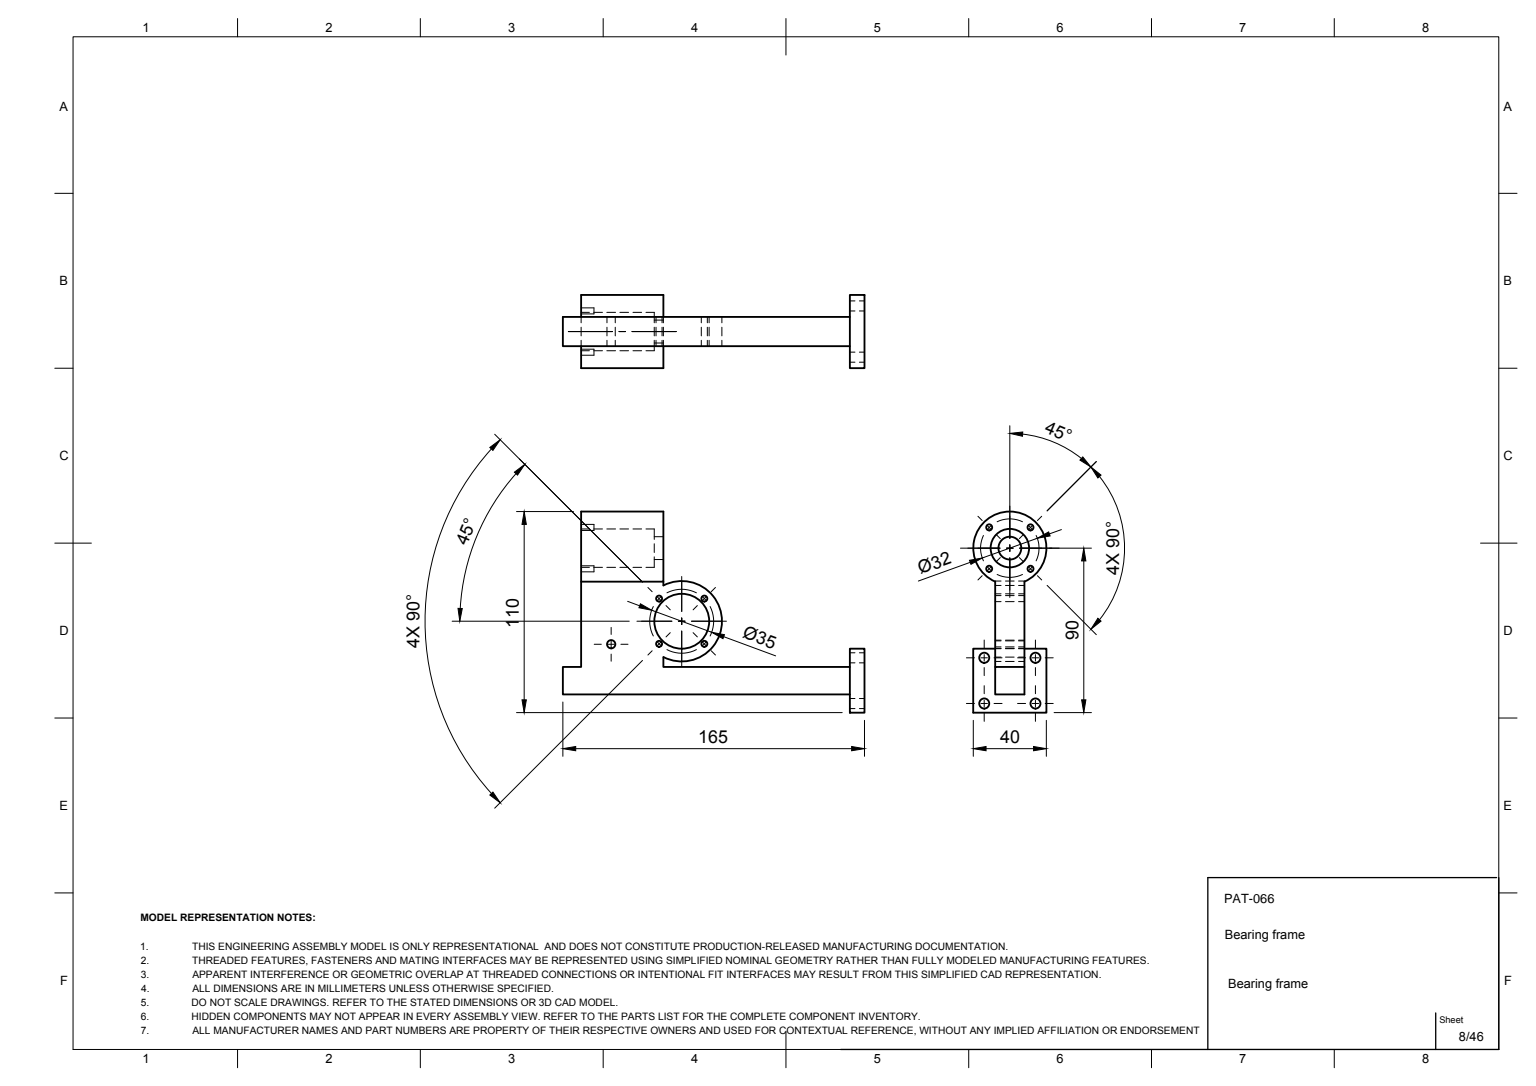
ISO-10303-21;
HEADER;
/* Generated by software containing ST-Developer
 * from STEP Tools, Inc. (www.steptools.com) 
 */

FILE_DESCRIPTION(
/* description */ ('Lever-operated bar clamp (toggle)'),
/* implementation_level */ '2;1');

FILE_NAME(
/* name */ 'Bearing frame.step',
/* time_stamp */ '2026-10-28T03:25:02-07:00',
/* author */ (''),
/* organization */ (''),
/* preprocessor_version */ 'ST-DEVELOPER v20.2',
/* originating_system */ 'Autodesk Translation Framework v15.17.0.0',
/* authorisation */ '');

FILE_SCHEMA (('AUTOMOTIVE_DESIGN { 1 0 10303 214 3 1 1 }'));
ENDSEC;

DATA;
#10=MECHANICAL_DESIGN_GEOMETRIC_PRESENTATION_REPRESENTATION('',(#413),#12413);
#337=SHAPE_REPRESENTATION_RELATIONSHIP('SRR','None',#12576,#375);
#375=ADVANCED_BREP_SHAPE_REPRESENTATION('',(#460),#12373);
#413=STYLED_ITEM('',(#12869),#460);
#460=MANIFOLD_SOLID_BREP('Body1',#6572);
#516=FACE_BOUND('',#1355,.T.);
#517=FACE_BOUND('',#1360,.T.);
#518=FACE_BOUND('',#1361,.T.);
#519=FACE_BOUND('',#1362,.T.);
#520=FACE_BOUND('',#1363,.T.);
#521=FACE_BOUND('',#1364,.T.);
#522=FACE_BOUND('',#1365,.T.);
#523=FACE_BOUND('',#1367,.T.);
#524=FACE_BOUND('',#1368,.T.);
#525=FACE_BOUND('',#1369,.T.);
#526=FACE_BOUND('',#1370,.T.);
#527=FACE_BOUND('',#1371,.T.);
#528=FACE_BOUND('',#1373,.T.);
#529=FACE_BOUND('',#1374,.T.);
#530=FACE_BOUND('',#1375,.T.);
#531=FACE_BOUND('',#1376,.T.);
#532=FACE_BOUND('',#1377,.T.);
#533=FACE_BOUND('',#1385,.T.);
#534=FACE_BOUND('',#1386,.T.);
#535=FACE_BOUND('',#1387,.T.);
#536=FACE_BOUND('',#1388,.T.);
#537=FACE_BOUND('',#1389,.T.);
#538=FACE_BOUND('',#1390,.T.);
#539=FACE_BOUND('',#1393,.T.);
#540=FACE_BOUND('',#1398,.T.);
#541=FACE_BOUND('',#1399,.T.);
#542=FACE_BOUND('',#1400,.T.);
#543=FACE_BOUND('',#1401,.T.);
#669=PLANE('',#7093);
#670=PLANE('',#7097);
#671=PLANE('',#7101);
#672=PLANE('',#7105);
#673=PLANE('',#7133);
#674=PLANE('',#7143);
#675=PLANE('',#7145);
#676=PLANE('',#7146);
#677=PLANE('',#7147);
#678=PLANE('',#7148);
#679=PLANE('',#7149);
#680=PLANE('',#7150);
#681=PLANE('',#7151);
#682=PLANE('',#7154);
#683=PLANE('',#7155);
#684=PLANE('',#7156);
#685=PLANE('',#7157);
#686=PLANE('',#7158);
#687=PLANE('',#7159);
#688=PLANE('',#7160);
#914=FACE_OUTER_BOUND('',#1336,.T.);
#915=FACE_OUTER_BOUND('',#1337,.T.);
#916=FACE_OUTER_BOUND('',#1338,.T.);
#917=FACE_OUTER_BOUND('',#1339,.T.);
#918=FACE_OUTER_BOUND('',#1340,.T.);
#919=FACE_OUTER_BOUND('',#1341,.T.);
#920=FACE_OUTER_BOUND('',#1342,.T.);
#921=FACE_OUTER_BOUND('',#1343,.T.);
#922=FACE_OUTER_BOUND('',#1344,.T.);
#923=FACE_OUTER_BOUND('',#1345,.T.);
#924=FACE_OUTER_BOUND('',#1346,.T.);
#925=FACE_OUTER_BOUND('',#1347,.T.);
#926=FACE_OUTER_BOUND('',#1348,.T.);
#927=FACE_OUTER_BOUND('',#1349,.T.);
#928=FACE_OUTER_BOUND('',#1350,.T.);
#929=FACE_OUTER_BOUND('',#1351,.T.);
#930=FACE_OUTER_BOUND('',#1352,.T.);
#931=FACE_OUTER_BOUND('',#1353,.T.);
#932=FACE_OUTER_BOUND('',#1354,.T.);
#933=FACE_OUTER_BOUND('',#1356,.T.);
#934=FACE_OUTER_BOUND('',#1357,.T.);
#935=FACE_OUTER_BOUND('',#1358,.T.);
#936=FACE_OUTER_BOUND('',#1359,.T.);
#937=FACE_OUTER_BOUND('',#1366,.T.);
#938=FACE_OUTER_BOUND('',#1372,.T.);
#939=FACE_OUTER_BOUND('',#1378,.T.);
#940=FACE_OUTER_BOUND('',#1379,.T.);
#941=FACE_OUTER_BOUND('',#1380,.T.);
#942=FACE_OUTER_BOUND('',#1381,.T.);
#943=FACE_OUTER_BOUND('',#1382,.T.);
#944=FACE_OUTER_BOUND('',#1383,.T.);
#945=FACE_OUTER_BOUND('',#1384,.T.);
#946=FACE_OUTER_BOUND('',#1391,.T.);
#947=FACE_OUTER_BOUND('',#1392,.T.);
#948=FACE_OUTER_BOUND('',#1394,.T.);
#949=FACE_OUTER_BOUND('',#1395,.T.);
#950=FACE_OUTER_BOUND('',#1396,.T.);
#951=FACE_OUTER_BOUND('',#1397,.T.);
#1336=EDGE_LOOP('',(#4541,#4542,#4543,#4544));
#1337=EDGE_LOOP('',(#4545,#4546,#4547,#4548));
#1338=EDGE_LOOP('',(#4549));
#1339=EDGE_LOOP('',(#4550,#4551,#4552,#4553));
#1340=EDGE_LOOP('',(#4554));
#1341=EDGE_LOOP('',(#4555,#4556,#4557,#4558));
#1342=EDGE_LOOP('',(#4559));
#1343=EDGE_LOOP('',(#4560,#4561,#4562,#4563));
#1344=EDGE_LOOP('',(#4564));
#1345=EDGE_LOOP('',(#4565,#4566,#4567,#4568));
#1346=EDGE_LOOP('',(#4569,#4570,#4571,#4572));
#1347=EDGE_LOOP('',(#4573,#4574,#4575,#4576));
#1348=EDGE_LOOP('',(#4577,#4578,#4579,#4580));
#1349=EDGE_LOOP('',(#4581,#4582,#4583,#4584));
#1350=EDGE_LOOP('',(#4585,#4586,#4587,#4588));
#1351=EDGE_LOOP('',(#4589,#4590,#4591,#4592));
#1352=EDGE_LOOP('',(#4593,#4594,#4595,#4596));
#1353=EDGE_LOOP('',(#4597,#4598,#4599,#4600));
#1354=EDGE_LOOP('',(#4601));
#1355=EDGE_LOOP('',(#4602));
#1356=EDGE_LOOP('',(#4603,#4604,#4605,#4606));
#1357=EDGE_LOOP('',(#4607,#4608,#4609,#4610));
#1358=EDGE_LOOP('',(#4611,#4612,#4613,#4614));
#1359=EDGE_LOOP('',(#4615,#4616,#4617,#4618,#4619,#4620,#4621,#4622,#4623,
#4624));
#1360=EDGE_LOOP('',(#4625));
#1361=EDGE_LOOP('',(#4626));
#1362=EDGE_LOOP('',(#4627));
#1363=EDGE_LOOP('',(#4628));
#1364=EDGE_LOOP('',(#4629));
#1365=EDGE_LOOP('',(#4630));
#1366=EDGE_LOOP('',(#4631,#4632,#4633,#4634));
#1367=EDGE_LOOP('',(#4635));
#1368=EDGE_LOOP('',(#4636));
#1369=EDGE_LOOP('',(#4637));
#1370=EDGE_LOOP('',(#4638));
#1371=EDGE_LOOP('',(#4639));
#1372=EDGE_LOOP('',(#4640,#4641,#4642,#4643));
#1373=EDGE_LOOP('',(#4644,#4645,#4646,#4647));
#1374=EDGE_LOOP('',(#4648));
#1375=EDGE_LOOP('',(#4649));
#1376=EDGE_LOOP('',(#4650));
#1377=EDGE_LOOP('',(#4651));
#1378=EDGE_LOOP('',(#4652,#4653,#4654,#4655));
#1379=EDGE_LOOP('',(#4656,#4657,#4658,#4659));
#1380=EDGE_LOOP('',(#4660,#4661,#4662,#4663));
#1381=EDGE_LOOP('',(#4664,#4665,#4666,#4667));
#1382=EDGE_LOOP('',(#4668,#4669,#4670,#4671));
#1383=EDGE_LOOP('',(#4672,#4673,#4674,#4675));
#1384=EDGE_LOOP('',(#4676,#4677,#4678,#4679,#4680,#4681,#4682,#4683,#4684,
#4685));
#1385=EDGE_LOOP('',(#4686));
#1386=EDGE_LOOP('',(#4687));
#1387=EDGE_LOOP('',(#4688));
#1388=EDGE_LOOP('',(#4689));
#1389=EDGE_LOOP('',(#4690));
#1390=EDGE_LOOP('',(#4691));
#1391=EDGE_LOOP('',(#4692,#4693,#4694,#4695));
#1392=EDGE_LOOP('',(#4696,#4697,#4698,#4699));
#1393=EDGE_LOOP('',(#4700));
#1394=EDGE_LOOP('',(#4701,#4702,#4703,#4704));
#1395=EDGE_LOOP('',(#4705,#4706,#4707,#4708));
#1396=EDGE_LOOP('',(#4709,#4710,#4711,#4712));
#1397=EDGE_LOOP('',(#4713,#4714,#4715,#4716));
#1398=EDGE_LOOP('',(#4717));
#1399=EDGE_LOOP('',(#4718));
#1400=EDGE_LOOP('',(#4719));
#1401=EDGE_LOOP('',(#4720));
#1895=LINE('',#10181,#2336);
#1896=LINE('',#10187,#2337);
#1897=LINE('',#10194,#2338);
#1898=LINE('',#10201,#2339);
#1899=LINE('',#10208,#2340);
#1900=LINE('',#10215,#2341);
#1901=LINE('',#10221,#2342);
#1902=LINE('',#10227,#2343);
#1903=LINE('',#10233,#2344);
#1904=LINE('',#10239,#2345);
#1905=LINE('',#10245,#2346);
#1906=LINE('',#10251,#2347);
#1907=LINE('',#10257,#2348);
#1908=LINE('',#10263,#2349);
#1909=LINE('',#10271,#2350);
#1910=LINE('',#10276,#2351);
#1911=LINE('',#10281,#2352);
#1912=LINE('',#10285,#2353);
#1913=LINE('',#10289,#2354);
#1914=LINE('',#10291,#2355);
#1915=LINE('',#10293,#2356);
#1916=LINE('',#10295,#2357);
#1917=LINE('',#10297,#2358);
#1918=LINE('',#10299,#2359);
#1919=LINE('',#10301,#2360);
#1920=LINE('',#10304,#2361);
#1921=LINE('',#10307,#2362);
#1922=LINE('',#10308,#2363);
#1923=LINE('',#10312,#2364);
#1924=LINE('',#10314,#2365);
#1925=LINE('',#10316,#2366);
#1926=LINE('',#10317,#2367);
#1927=LINE('',#10320,#2368);
#1928=LINE('',#10321,#2369);
#1929=LINE('',#10322,#2370);
#1930=LINE('',#10326,#2371);
#1931=LINE('',#10327,#2372);
#1932=LINE('',#10328,#2373);
#1933=LINE('',#10331,#2374);
#1934=LINE('',#10332,#2375);
#1935=LINE('',#10335,#2376);
#1936=LINE('',#10336,#2377);
#1937=LINE('',#10338,#2378);
#1938=LINE('',#10341,#2379);
#1939=LINE('',#10342,#2380);
#1940=LINE('',#10345,#2381);
#1941=LINE('',#10347,#2382);
#1942=LINE('',#10350,#2383);
#1943=LINE('',#10351,#2384);
#1944=LINE('',#10353,#2385);
#1945=LINE('',#10355,#2386);
#1946=LINE('',#10356,#2387);
#1947=LINE('',#10360,#2388);
#1948=LINE('',#10362,#2389);
#2336=VECTOR('',#8038,0.225);
#2337=VECTOR('',#8045,0.165);
#2338=VECTOR('',#8054,0.165);
#2339=VECTOR('',#8063,0.165);
#2340=VECTOR('',#8072,0.165);
#2341=VECTOR('',#8081,0.165);
#2342=VECTOR('',#8088,0.165);
#2343=VECTOR('',#8095,0.165);
#2344=VECTOR('',#8102,0.165);
#2345=VECTOR('',#8109,0.275);
#2346=VECTOR('',#8116,0.275);
#2347=VECTOR('',#8123,0.275);
#2348=VECTOR('',#8130,0.275);
#2349=VECTOR('',#8137,1.05);
#2350=VECTOR('',#8148,0.625);
#2351=VECTOR('',#8153,1.5);
#2352=VECTOR('',#8158,1.);
#2353=VECTOR('',#8161,1.);
#2354=VECTOR('',#8166,1.);
#2355=VECTOR('',#8167,1.);
#2356=VECTOR('',#8168,1.);
#2357=VECTOR('',#8169,1.);
#2358=VECTOR('',#8170,1.);
#2359=VECTOR('',#8171,1.);
#2360=VECTOR('',#8172,1.);
#2361=VECTOR('',#8175,1.);
#2362=VECTOR('',#8178,1.);
#2363=VECTOR('',#8179,1.);
#2364=VECTOR('',#8182,1.);
#2365=VECTOR('',#8183,1.);
#2366=VECTOR('',#8184,1.);
#2367=VECTOR('',#8185,1.);
#2368=VECTOR('',#8186,1.);
#2369=VECTOR('',#8187,1.);
#2370=VECTOR('',#8188,1.);
#2371=VECTOR('',#8191,1.);
#2372=VECTOR('',#8192,1.);
#2373=VECTOR('',#8193,1.);
#2374=VECTOR('',#8196,1.);
#2375=VECTOR('',#8197,1.);
#2376=VECTOR('',#8200,1.);
#2377=VECTOR('',#8201,1.);
#2378=VECTOR('',#8204,1.);
#2379=VECTOR('',#8207,1.);
#2380=VECTOR('',#8208,1.);
#2381=VECTOR('',#8211,1.);
#2382=VECTOR('',#8212,1.);
#2383=VECTOR('',#8217,1.);
#2384=VECTOR('',#8218,1.);
#2385=VECTOR('',#8219,1.);
#2386=VECTOR('',#8220,1.);
#2387=VECTOR('',#8221,1.);
#2388=VECTOR('',#8228,1.);
#2389=VECTOR('',#8231,1.);
#2749=CIRCLE('',#7088,0.225);
#2750=CIRCLE('',#7089,0.225);
#2751=CIRCLE('',#7091,0.165);
#2752=CIRCLE('',#7092,0.165);
#2753=CIRCLE('',#7095,0.165);
#2754=CIRCLE('',#7096,0.165);
#2755=CIRCLE('',#7099,0.165);
#2756=CIRCLE('',#7100,0.165);
#2757=CIRCLE('',#7103,0.165);
#2758=CIRCLE('',#7104,0.165);
#2759=CIRCLE('',#7107,0.165);
#2760=CIRCLE('',#7108,0.165);
#2761=CIRCLE('',#7110,0.165);
#2762=CIRCLE('',#7111,0.165);
#2763=CIRCLE('',#7113,0.165);
#2764=CIRCLE('',#7114,0.165);
#2765=CIRCLE('',#7116,0.165);
#2766=CIRCLE('',#7117,0.165);
#2767=CIRCLE('',#7119,0.275);
#2768=CIRCLE('',#7120,0.275);
#2769=CIRCLE('',#7122,0.275);
#2770=CIRCLE('',#7123,0.275);
#2771=CIRCLE('',#7125,0.275);
#2772=CIRCLE('',#7126,0.275);
#2773=CIRCLE('',#7128,0.275);
#2774=CIRCLE('',#7129,0.275);
#2775=CIRCLE('',#7131,1.05);
#2776=CIRCLE('',#7132,1.05);
#2777=CIRCLE('',#7134,0.625);
#2778=CIRCLE('',#7136,0.625);
#2779=CIRCLE('',#7138,1.5);
#2780=CIRCLE('',#7139,1.5);
#2781=CIRCLE('',#7141,2.);
#2782=CIRCLE('',#7142,2.);
#2783=CIRCLE('',#7144,2.2);
#2784=CIRCLE('',#7153,2.2);
#3114=VERTEX_POINT('',#10178);
#3115=VERTEX_POINT('',#10180);
#3116=VERTEX_POINT('',#10184);
#3117=VERTEX_POINT('',#10186);
#3118=VERTEX_POINT('',#10191);
#3119=VERTEX_POINT('',#10193);
#3120=VERTEX_POINT('',#10198);
#3121=VERTEX_POINT('',#10200);
#3122=VERTEX_POINT('',#10205);
#3123=VERTEX_POINT('',#10207);
#3124=VERTEX_POINT('',#10212);
#3125=VERTEX_POINT('',#10214);
#3126=VERTEX_POINT('',#10218);
#3127=VERTEX_POINT('',#10220);
#3128=VERTEX_POINT('',#10224);
#3129=VERTEX_POINT('',#10226);
#3130=VERTEX_POINT('',#10230);
#3131=VERTEX_POINT('',#10232);
#3132=VERTEX_POINT('',#10236);
#3133=VERTEX_POINT('',#10238);
#3134=VERTEX_POINT('',#10242);
#3135=VERTEX_POINT('',#10244);
#3136=VERTEX_POINT('',#10248);
#3137=VERTEX_POINT('',#10250);
#3138=VERTEX_POINT('',#10254);
#3139=VERTEX_POINT('',#10256);
#3140=VERTEX_POINT('',#10260);
#3141=VERTEX_POINT('',#10262);
#3142=VERTEX_POINT('',#10266);
#3143=VERTEX_POINT('',#10269);
#3144=VERTEX_POINT('',#10273);
#3145=VERTEX_POINT('',#10275);
#3146=VERTEX_POINT('',#10279);
#3147=VERTEX_POINT('',#10280);
#3148=VERTEX_POINT('',#10282);
#3149=VERTEX_POINT('',#10284);
#3150=VERTEX_POINT('',#10288);
#3151=VERTEX_POINT('',#10290);
#3152=VERTEX_POINT('',#10292);
#3153=VERTEX_POINT('',#10294);
#3154=VERTEX_POINT('',#10296);
#3155=VERTEX_POINT('',#10298);
#3156=VERTEX_POINT('',#10300);
#3157=VERTEX_POINT('',#10302);
#3158=VERTEX_POINT('',#10306);
#3159=VERTEX_POINT('',#10310);
#3160=VERTEX_POINT('',#10311);
#3161=VERTEX_POINT('',#10313);
#3162=VERTEX_POINT('',#10315);
#3163=VERTEX_POINT('',#10318);
#3164=VERTEX_POINT('',#10319);
#3165=VERTEX_POINT('',#10324);
#3166=VERTEX_POINT('',#10325);
#3167=VERTEX_POINT('',#10330);
#3168=VERTEX_POINT('',#10334);
#3169=VERTEX_POINT('',#10340);
#3170=VERTEX_POINT('',#10344);
#3171=VERTEX_POINT('',#10346);
#3172=VERTEX_POINT('',#10352);
#3173=VERTEX_POINT('',#10354);
#3675=EDGE_CURVE('',#3114,#3114,#2749,.T.);
#3676=EDGE_CURVE('',#3114,#3115,#1895,.T.);
#3677=EDGE_CURVE('',#3115,#3115,#2750,.T.);
#3678=EDGE_CURVE('',#3116,#3116,#2751,.T.);
#3679=EDGE_CURVE('',#3116,#3117,#1896,.T.);
#3680=EDGE_CURVE('',#3117,#3117,#2752,.T.);
#3681=EDGE_CURVE('',#3118,#3118,#2753,.T.);
#3682=EDGE_CURVE('',#3118,#3119,#1897,.T.);
#3683=EDGE_CURVE('',#3119,#3119,#2754,.T.);
#3684=EDGE_CURVE('',#3120,#3120,#2755,.T.);
#3685=EDGE_CURVE('',#3120,#3121,#1898,.T.);
#3686=EDGE_CURVE('',#3121,#3121,#2756,.T.);
#3687=EDGE_CURVE('',#3122,#3122,#2757,.T.);
#3688=EDGE_CURVE('',#3122,#3123,#1899,.T.);
#3689=EDGE_CURVE('',#3123,#3123,#2758,.T.);
#3690=EDGE_CURVE('',#3124,#3124,#2759,.T.);
#3691=EDGE_CURVE('',#3124,#3125,#1900,.T.);
#3692=EDGE_CURVE('',#3125,#3125,#2760,.T.);
#3693=EDGE_CURVE('',#3126,#3126,#2761,.T.);
#3694=EDGE_CURVE('',#3126,#3127,#1901,.T.);
#3695=EDGE_CURVE('',#3127,#3127,#2762,.T.);
#3696=EDGE_CURVE('',#3128,#3128,#2763,.T.);
#3697=EDGE_CURVE('',#3128,#3129,#1902,.T.);
#3698=EDGE_CURVE('',#3129,#3129,#2764,.T.);
#3699=EDGE_CURVE('',#3130,#3130,#2765,.T.);
#3700=EDGE_CURVE('',#3130,#3131,#1903,.T.);
#3701=EDGE_CURVE('',#3131,#3131,#2766,.T.);
#3702=EDGE_CURVE('',#3132,#3132,#2767,.T.);
#3703=EDGE_CURVE('',#3132,#3133,#1904,.T.);
#3704=EDGE_CURVE('',#3133,#3133,#2768,.T.);
#3705=EDGE_CURVE('',#3134,#3134,#2769,.T.);
#3706=EDGE_CURVE('',#3134,#3135,#1905,.T.);
#3707=EDGE_CURVE('',#3135,#3135,#2770,.T.);
#3708=EDGE_CURVE('',#3136,#3136,#2771,.T.);
#3709=EDGE_CURVE('',#3136,#3137,#1906,.T.);
#3710=EDGE_CURVE('',#3137,#3137,#2772,.T.);
#3711=EDGE_CURVE('',#3138,#3138,#2773,.T.);
#3712=EDGE_CURVE('',#3138,#3139,#1907,.T.);
#3713=EDGE_CURVE('',#3139,#3139,#2774,.T.);
#3714=EDGE_CURVE('',#3140,#3140,#2775,.T.);
#3715=EDGE_CURVE('',#3140,#3141,#1908,.T.);
#3716=EDGE_CURVE('',#3141,#3141,#2776,.T.);
#3717=EDGE_CURVE('',#3142,#3142,#2777,.T.);
#3718=EDGE_CURVE('',#3143,#3143,#2778,.T.);
#3719=EDGE_CURVE('',#3143,#3142,#1909,.T.);
#3720=EDGE_CURVE('',#3144,#3144,#2779,.T.);
#3721=EDGE_CURVE('',#3144,#3145,#1910,.T.);
#3722=EDGE_CURVE('',#3145,#3145,#2780,.T.);
#3723=EDGE_CURVE('',#3146,#3147,#1911,.T.);
#3724=EDGE_CURVE('',#3146,#3148,#2781,.T.);
#3725=EDGE_CURVE('',#3149,#3148,#1912,.T.);
#3726=EDGE_CURVE('',#3147,#3149,#2782,.T.);
#3727=EDGE_CURVE('',#3147,#3150,#1913,.T.);
#3728=EDGE_CURVE('',#3150,#3151,#1914,.T.);
#3729=EDGE_CURVE('',#3152,#3151,#1915,.T.);
#3730=EDGE_CURVE('',#3153,#3152,#1916,.T.);
#3731=EDGE_CURVE('',#3153,#3154,#1917,.T.);
#3732=EDGE_CURVE('',#3154,#3155,#1918,.T.);
#3733=EDGE_CURVE('',#3155,#3156,#1919,.T.);
#3734=EDGE_CURVE('',#3157,#3156,#2783,.T.);
#3735=EDGE_CURVE('',#3157,#3146,#1920,.T.);
#3736=EDGE_CURVE('',#3158,#3149,#1921,.T.);
#3737=EDGE_CURVE('',#3150,#3158,#1922,.T.);
#3738=EDGE_CURVE('',#3159,#3160,#1923,.T.);
#3739=EDGE_CURVE('',#3160,#3161,#1924,.T.);
#3740=EDGE_CURVE('',#3161,#3162,#1925,.T.);
#3741=EDGE_CURVE('',#3162,#3159,#1926,.T.);
#3742=EDGE_CURVE('',#3163,#3164,#1927,.T.);
#3743=EDGE_CURVE('',#3154,#3163,#1928,.T.);
#3744=EDGE_CURVE('',#3164,#3153,#1929,.T.);
#3745=EDGE_CURVE('',#3165,#3166,#1930,.T.);
#3746=EDGE_CURVE('',#3166,#3159,#1931,.T.);
#3747=EDGE_CURVE('',#3165,#3162,#1932,.T.);
#3748=EDGE_CURVE('',#3167,#3165,#1933,.T.);
#3749=EDGE_CURVE('',#3167,#3161,#1934,.T.);
#3750=EDGE_CURVE('',#3168,#3167,#1935,.T.);
#3751=EDGE_CURVE('',#3168,#3160,#1936,.T.);
#3752=EDGE_CURVE('',#3166,#3168,#1937,.T.);
#3753=EDGE_CURVE('',#3163,#3169,#1938,.T.);
#3754=EDGE_CURVE('',#3169,#3155,#1939,.T.);
#3755=EDGE_CURVE('',#3157,#3170,#1940,.T.);
#3756=EDGE_CURVE('',#3171,#3156,#1941,.T.);
#3757=EDGE_CURVE('',#3170,#3171,#2784,.T.);
#3758=EDGE_CURVE('',#3148,#3170,#1942,.T.);
#3759=EDGE_CURVE('',#3171,#3169,#1943,.T.);
#3760=EDGE_CURVE('',#3164,#3172,#1944,.T.);
#3761=EDGE_CURVE('',#3173,#3172,#1945,.T.);
#3762=EDGE_CURVE('',#3158,#3173,#1946,.T.);
#3763=EDGE_CURVE('',#3151,#3173,#1947,.T.);
#3764=EDGE_CURVE('',#3172,#3152,#1948,.T.);
#4541=ORIENTED_EDGE('',*,*,#3675,.F.);
#4542=ORIENTED_EDGE('',*,*,#3676,.T.);
#4543=ORIENTED_EDGE('',*,*,#3677,.F.);
#4544=ORIENTED_EDGE('',*,*,#3676,.F.);
#4545=ORIENTED_EDGE('',*,*,#3678,.F.);
#4546=ORIENTED_EDGE('',*,*,#3679,.T.);
#4547=ORIENTED_EDGE('',*,*,#3680,.F.);
#4548=ORIENTED_EDGE('',*,*,#3679,.F.);
#4549=ORIENTED_EDGE('',*,*,#3678,.T.);
#4550=ORIENTED_EDGE('',*,*,#3681,.F.);
#4551=ORIENTED_EDGE('',*,*,#3682,.T.);
#4552=ORIENTED_EDGE('',*,*,#3683,.F.);
#4553=ORIENTED_EDGE('',*,*,#3682,.F.);
#4554=ORIENTED_EDGE('',*,*,#3681,.T.);
#4555=ORIENTED_EDGE('',*,*,#3684,.F.);
#4556=ORIENTED_EDGE('',*,*,#3685,.T.);
#4557=ORIENTED_EDGE('',*,*,#3686,.F.);
#4558=ORIENTED_EDGE('',*,*,#3685,.F.);
#4559=ORIENTED_EDGE('',*,*,#3684,.T.);
#4560=ORIENTED_EDGE('',*,*,#3687,.F.);
#4561=ORIENTED_EDGE('',*,*,#3688,.T.);
#4562=ORIENTED_EDGE('',*,*,#3689,.F.);
#4563=ORIENTED_EDGE('',*,*,#3688,.F.);
#4564=ORIENTED_EDGE('',*,*,#3687,.T.);
#4565=ORIENTED_EDGE('',*,*,#3690,.F.);
#4566=ORIENTED_EDGE('',*,*,#3691,.T.);
#4567=ORIENTED_EDGE('',*,*,#3692,.F.);
#4568=ORIENTED_EDGE('',*,*,#3691,.F.);
#4569=ORIENTED_EDGE('',*,*,#3693,.F.);
#4570=ORIENTED_EDGE('',*,*,#3694,.T.);
#4571=ORIENTED_EDGE('',*,*,#3695,.F.);
#4572=ORIENTED_EDGE('',*,*,#3694,.F.);
#4573=ORIENTED_EDGE('',*,*,#3696,.F.);
#4574=ORIENTED_EDGE('',*,*,#3697,.T.);
#4575=ORIENTED_EDGE('',*,*,#3698,.F.);
#4576=ORIENTED_EDGE('',*,*,#3697,.F.);
#4577=ORIENTED_EDGE('',*,*,#3699,.F.);
#4578=ORIENTED_EDGE('',*,*,#3700,.T.);
#4579=ORIENTED_EDGE('',*,*,#3701,.F.);
#4580=ORIENTED_EDGE('',*,*,#3700,.F.);
#4581=ORIENTED_EDGE('',*,*,#3702,.F.);
#4582=ORIENTED_EDGE('',*,*,#3703,.T.);
#4583=ORIENTED_EDGE('',*,*,#3704,.F.);
#4584=ORIENTED_EDGE('',*,*,#3703,.F.);
#4585=ORIENTED_EDGE('',*,*,#3705,.F.);
#4586=ORIENTED_EDGE('',*,*,#3706,.T.);
#4587=ORIENTED_EDGE('',*,*,#3707,.F.);
#4588=ORIENTED_EDGE('',*,*,#3706,.F.);
#4589=ORIENTED_EDGE('',*,*,#3708,.F.);
#4590=ORIENTED_EDGE('',*,*,#3709,.T.);
#4591=ORIENTED_EDGE('',*,*,#3710,.F.);
#4592=ORIENTED_EDGE('',*,*,#3709,.F.);
#4593=ORIENTED_EDGE('',*,*,#3711,.F.);
#4594=ORIENTED_EDGE('',*,*,#3712,.T.);
#4595=ORIENTED_EDGE('',*,*,#3713,.F.);
#4596=ORIENTED_EDGE('',*,*,#3712,.F.);
#4597=ORIENTED_EDGE('',*,*,#3714,.F.);
#4598=ORIENTED_EDGE('',*,*,#3715,.T.);
#4599=ORIENTED_EDGE('',*,*,#3716,.F.);
#4600=ORIENTED_EDGE('',*,*,#3715,.F.);
#4601=ORIENTED_EDGE('',*,*,#3714,.T.);
#4602=ORIENTED_EDGE('',*,*,#3717,.F.);
#4603=ORIENTED_EDGE('',*,*,#3718,.F.);
#4604=ORIENTED_EDGE('',*,*,#3719,.T.);
#4605=ORIENTED_EDGE('',*,*,#3717,.T.);
#4606=ORIENTED_EDGE('',*,*,#3719,.F.);
#4607=ORIENTED_EDGE('',*,*,#3720,.F.);
#4608=ORIENTED_EDGE('',*,*,#3721,.T.);
#4609=ORIENTED_EDGE('',*,*,#3722,.F.);
#4610=ORIENTED_EDGE('',*,*,#3721,.F.);
#4611=ORIENTED_EDGE('',*,*,#3723,.F.);
#4612=ORIENTED_EDGE('',*,*,#3724,.T.);
#4613=ORIENTED_EDGE('',*,*,#3725,.F.);
#4614=ORIENTED_EDGE('',*,*,#3726,.F.);
#4615=ORIENTED_EDGE('',*,*,#3723,.T.);
#4616=ORIENTED_EDGE('',*,*,#3727,.T.);
#4617=ORIENTED_EDGE('',*,*,#3728,.T.);
#4618=ORIENTED_EDGE('',*,*,#3729,.F.);
#4619=ORIENTED_EDGE('',*,*,#3730,.F.);
#4620=ORIENTED_EDGE('',*,*,#3731,.T.);
#4621=ORIENTED_EDGE('',*,*,#3732,.T.);
#4622=ORIENTED_EDGE('',*,*,#3733,.T.);
#4623=ORIENTED_EDGE('',*,*,#3734,.F.);
#4624=ORIENTED_EDGE('',*,*,#3735,.T.);
#4625=ORIENTED_EDGE('',*,*,#3675,.T.);
#4626=ORIENTED_EDGE('',*,*,#3720,.T.);
#4627=ORIENTED_EDGE('',*,*,#3699,.T.);
#4628=ORIENTED_EDGE('',*,*,#3696,.T.);
#4629=ORIENTED_EDGE('',*,*,#3693,.T.);
#4630=ORIENTED_EDGE('',*,*,#3690,.T.);
#4631=ORIENTED_EDGE('',*,*,#3726,.T.);
#4632=ORIENTED_EDGE('',*,*,#3736,.F.);
#4633=ORIENTED_EDGE('',*,*,#3737,.F.);
#4634=ORIENTED_EDGE('',*,*,#3727,.F.);
#4635=ORIENTED_EDGE('',*,*,#3716,.T.);
#4636=ORIENTED_EDGE('',*,*,#3689,.T.);
#4637=ORIENTED_EDGE('',*,*,#3686,.T.);
#4638=ORIENTED_EDGE('',*,*,#3683,.T.);
#4639=ORIENTED_EDGE('',*,*,#3680,.T.);
#4640=ORIENTED_EDGE('',*,*,#3738,.T.);
#4641=ORIENTED_EDGE('',*,*,#3739,.T.);
#4642=ORIENTED_EDGE('',*,*,#3740,.T.);
#4643=ORIENTED_EDGE('',*,*,#3741,.T.);
#4644=ORIENTED_EDGE('',*,*,#3742,.F.);
#4645=ORIENTED_EDGE('',*,*,#3743,.F.);
#4646=ORIENTED_EDGE('',*,*,#3731,.F.);
#4647=ORIENTED_EDGE('',*,*,#3744,.F.);
#4648=ORIENTED_EDGE('',*,*,#3713,.T.);
#4649=ORIENTED_EDGE('',*,*,#3710,.T.);
#4650=ORIENTED_EDGE('',*,*,#3707,.T.);
#4651=ORIENTED_EDGE('',*,*,#3704,.T.);
#4652=ORIENTED_EDGE('',*,*,#3745,.T.);
#4653=ORIENTED_EDGE('',*,*,#3746,.T.);
#4654=ORIENTED_EDGE('',*,*,#3741,.F.);
#4655=ORIENTED_EDGE('',*,*,#3747,.F.);
#4656=ORIENTED_EDGE('',*,*,#3748,.T.);
#4657=ORIENTED_EDGE('',*,*,#3747,.T.);
#4658=ORIENTED_EDGE('',*,*,#3740,.F.);
#4659=ORIENTED_EDGE('',*,*,#3749,.F.);
#4660=ORIENTED_EDGE('',*,*,#3750,.T.);
#4661=ORIENTED_EDGE('',*,*,#3749,.T.);
#4662=ORIENTED_EDGE('',*,*,#3739,.F.);
#4663=ORIENTED_EDGE('',*,*,#3751,.F.);
#4664=ORIENTED_EDGE('',*,*,#3752,.T.);
#4665=ORIENTED_EDGE('',*,*,#3751,.T.);
#4666=ORIENTED_EDGE('',*,*,#3738,.F.);
#4667=ORIENTED_EDGE('',*,*,#3746,.F.);
#4668=ORIENTED_EDGE('',*,*,#3743,.T.);
#4669=ORIENTED_EDGE('',*,*,#3753,.T.);
#4670=ORIENTED_EDGE('',*,*,#3754,.T.);
#4671=ORIENTED_EDGE('',*,*,#3732,.F.);
#4672=ORIENTED_EDGE('',*,*,#3755,.F.);
#4673=ORIENTED_EDGE('',*,*,#3734,.T.);
#4674=ORIENTED_EDGE('',*,*,#3756,.F.);
#4675=ORIENTED_EDGE('',*,*,#3757,.F.);
#4676=ORIENTED_EDGE('',*,*,#3725,.T.);
#4677=ORIENTED_EDGE('',*,*,#3758,.T.);
#4678=ORIENTED_EDGE('',*,*,#3757,.T.);
#4679=ORIENTED_EDGE('',*,*,#3759,.T.);
#4680=ORIENTED_EDGE('',*,*,#3753,.F.);
#4681=ORIENTED_EDGE('',*,*,#3742,.T.);
#4682=ORIENTED_EDGE('',*,*,#3760,.T.);
#4683=ORIENTED_EDGE('',*,*,#3761,.F.);
#4684=ORIENTED_EDGE('',*,*,#3762,.F.);
#4685=ORIENTED_EDGE('',*,*,#3736,.T.);
#4686=ORIENTED_EDGE('',*,*,#3677,.T.);
#4687=ORIENTED_EDGE('',*,*,#3722,.T.);
#4688=ORIENTED_EDGE('',*,*,#3701,.T.);
#4689=ORIENTED_EDGE('',*,*,#3698,.T.);
#4690=ORIENTED_EDGE('',*,*,#3695,.T.);
#4691=ORIENTED_EDGE('',*,*,#3692,.T.);
#4692=ORIENTED_EDGE('',*,*,#3756,.T.);
#4693=ORIENTED_EDGE('',*,*,#3733,.F.);
#4694=ORIENTED_EDGE('',*,*,#3754,.F.);
#4695=ORIENTED_EDGE('',*,*,#3759,.F.);
#4696=ORIENTED_EDGE('',*,*,#3735,.F.);
#4697=ORIENTED_EDGE('',*,*,#3755,.T.);
#4698=ORIENTED_EDGE('',*,*,#3758,.F.);
#4699=ORIENTED_EDGE('',*,*,#3724,.F.);
#4700=ORIENTED_EDGE('',*,*,#3718,.T.);
#4701=ORIENTED_EDGE('',*,*,#3737,.T.);
#4702=ORIENTED_EDGE('',*,*,#3762,.T.);
#4703=ORIENTED_EDGE('',*,*,#3763,.F.);
#4704=ORIENTED_EDGE('',*,*,#3728,.F.);
#4705=ORIENTED_EDGE('',*,*,#3744,.T.);
#4706=ORIENTED_EDGE('',*,*,#3730,.T.);
#4707=ORIENTED_EDGE('',*,*,#3764,.F.);
#4708=ORIENTED_EDGE('',*,*,#3760,.F.);
#4709=ORIENTED_EDGE('',*,*,#3764,.T.);
#4710=ORIENTED_EDGE('',*,*,#3729,.T.);
#4711=ORIENTED_EDGE('',*,*,#3763,.T.);
#4712=ORIENTED_EDGE('',*,*,#3761,.T.);
#4713=ORIENTED_EDGE('',*,*,#3752,.F.);
#4714=ORIENTED_EDGE('',*,*,#3745,.F.);
#4715=ORIENTED_EDGE('',*,*,#3748,.F.);
#4716=ORIENTED_EDGE('',*,*,#3750,.F.);
#4717=ORIENTED_EDGE('',*,*,#3702,.T.);
#4718=ORIENTED_EDGE('',*,*,#3705,.T.);
#4719=ORIENTED_EDGE('',*,*,#3708,.T.);
#4720=ORIENTED_EDGE('',*,*,#3711,.T.);
#6041=CYLINDRICAL_SURFACE('',#7087,0.225);
#6042=CYLINDRICAL_SURFACE('',#7090,0.165);
#6043=CYLINDRICAL_SURFACE('',#7094,0.165);
#6044=CYLINDRICAL_SURFACE('',#7098,0.165);
#6045=CYLINDRICAL_SURFACE('',#7102,0.165);
#6046=CYLINDRICAL_SURFACE('',#7106,0.165);
#6047=CYLINDRICAL_SURFACE('',#7109,0.165);
#6048=CYLINDRICAL_SURFACE('',#7112,0.165);
#6049=CYLINDRICAL_SURFACE('',#7115,0.165);
#6050=CYLINDRICAL_SURFACE('',#7118,0.275);
#6051=CYLINDRICAL_SURFACE('',#7121,0.275);
#6052=CYLINDRICAL_SURFACE('',#7124,0.275);
#6053=CYLINDRICAL_SURFACE('',#7127,0.275);
#6054=CYLINDRICAL_SURFACE('',#7130,1.05);
#6055=CYLINDRICAL_SURFACE('',#7135,0.625);
#6056=CYLINDRICAL_SURFACE('',#7137,1.5);
#6057=CYLINDRICAL_SURFACE('',#7140,2.);
#6058=CYLINDRICAL_SURFACE('',#7152,2.2);
#6189=ADVANCED_FACE('',(#914),#6041,.F.);
#6190=ADVANCED_FACE('',(#915),#6042,.F.);
#6191=ADVANCED_FACE('',(#916),#669,.T.);
#6192=ADVANCED_FACE('',(#917),#6043,.F.);
#6193=ADVANCED_FACE('',(#918),#670,.T.);
#6194=ADVANCED_FACE('',(#919),#6044,.F.);
#6195=ADVANCED_FACE('',(#920),#671,.T.);
#6196=ADVANCED_FACE('',(#921),#6045,.F.);
#6197=ADVANCED_FACE('',(#922),#672,.T.);
#6198=ADVANCED_FACE('',(#923),#6046,.F.);
#6199=ADVANCED_FACE('',(#924),#6047,.F.);
#6200=ADVANCED_FACE('',(#925),#6048,.F.);
#6201=ADVANCED_FACE('',(#926),#6049,.F.);
#6202=ADVANCED_FACE('',(#927),#6050,.F.);
#6203=ADVANCED_FACE('',(#928),#6051,.F.);
#6204=ADVANCED_FACE('',(#929),#6052,.F.);
#6205=ADVANCED_FACE('',(#930),#6053,.F.);
#6206=ADVANCED_FACE('',(#931),#6054,.F.);
#6207=ADVANCED_FACE('',(#932,#516),#673,.T.);
#6208=ADVANCED_FACE('',(#933),#6055,.F.);
#6209=ADVANCED_FACE('',(#934),#6056,.F.);
#6210=ADVANCED_FACE('',(#935),#6057,.T.);
#6211=ADVANCED_FACE('',(#936,#517,#518,#519,#520,#521,#522),#674,.T.);
#6212=ADVANCED_FACE('',(#937,#523,#524,#525,#526,#527),#675,.T.);
#6213=ADVANCED_FACE('',(#938,#528,#529,#530,#531,#532),#676,.T.);
#6214=ADVANCED_FACE('',(#939),#677,.T.);
#6215=ADVANCED_FACE('',(#940),#678,.T.);
#6216=ADVANCED_FACE('',(#941),#679,.T.);
#6217=ADVANCED_FACE('',(#942),#680,.T.);
#6218=ADVANCED_FACE('',(#943),#681,.T.);
#6219=ADVANCED_FACE('',(#944),#6058,.T.);
#6220=ADVANCED_FACE('',(#945,#533,#534,#535,#536,#537,#538),#682,.T.);
#6221=ADVANCED_FACE('',(#946),#683,.T.);
#6222=ADVANCED_FACE('',(#947,#539),#684,.T.);
#6223=ADVANCED_FACE('',(#948),#685,.T.);
#6224=ADVANCED_FACE('',(#949),#686,.T.);
#6225=ADVANCED_FACE('',(#950),#687,.T.);
#6226=ADVANCED_FACE('',(#951,#540,#541,#542,#543),#688,.F.);
#6572=CLOSED_SHELL('',(#6189,#6190,#6191,#6192,#6193,#6194,#6195,#6196,
#6197,#6198,#6199,#6200,#6201,#6202,#6203,#6204,#6205,#6206,#6207,#6208,
#6209,#6210,#6211,#6212,#6213,#6214,#6215,#6216,#6217,#6218,#6219,#6220,
#6221,#6222,#6223,#6224,#6225,#6226));
#7086=AXIS2_PLACEMENT_3D('',#10176,#8032,#8033);
#7087=AXIS2_PLACEMENT_3D('',#10177,#8034,#8035);
#7088=AXIS2_PLACEMENT_3D('',#10179,#8036,#8037);
#7089=AXIS2_PLACEMENT_3D('',#10182,#8039,#8040);
#7090=AXIS2_PLACEMENT_3D('',#10183,#8041,#8042);
#7091=AXIS2_PLACEMENT_3D('',#10185,#8043,#8044);
#7092=AXIS2_PLACEMENT_3D('',#10188,#8046,#8047);
#7093=AXIS2_PLACEMENT_3D('',#10189,#8048,#8049);
#7094=AXIS2_PLACEMENT_3D('',#10190,#8050,#8051);
#7095=AXIS2_PLACEMENT_3D('',#10192,#8052,#8053);
#7096=AXIS2_PLACEMENT_3D('',#10195,#8055,#8056);
#7097=AXIS2_PLACEMENT_3D('',#10196,#8057,#8058);
#7098=AXIS2_PLACEMENT_3D('',#10197,#8059,#8060);
#7099=AXIS2_PLACEMENT_3D('',#10199,#8061,#8062);
#7100=AXIS2_PLACEMENT_3D('',#10202,#8064,#8065);
#7101=AXIS2_PLACEMENT_3D('',#10203,#8066,#8067);
#7102=AXIS2_PLACEMENT_3D('',#10204,#8068,#8069);
#7103=AXIS2_PLACEMENT_3D('',#10206,#8070,#8071);
#7104=AXIS2_PLACEMENT_3D('',#10209,#8073,#8074);
#7105=AXIS2_PLACEMENT_3D('',#10210,#8075,#8076);
#7106=AXIS2_PLACEMENT_3D('',#10211,#8077,#8078);
#7107=AXIS2_PLACEMENT_3D('',#10213,#8079,#8080);
#7108=AXIS2_PLACEMENT_3D('',#10216,#8082,#8083);
#7109=AXIS2_PLACEMENT_3D('',#10217,#8084,#8085);
#7110=AXIS2_PLACEMENT_3D('',#10219,#8086,#8087);
#7111=AXIS2_PLACEMENT_3D('',#10222,#8089,#8090);
#7112=AXIS2_PLACEMENT_3D('',#10223,#8091,#8092);
#7113=AXIS2_PLACEMENT_3D('',#10225,#8093,#8094);
#7114=AXIS2_PLACEMENT_3D('',#10228,#8096,#8097);
#7115=AXIS2_PLACEMENT_3D('',#10229,#8098,#8099);
#7116=AXIS2_PLACEMENT_3D('',#10231,#8100,#8101);
#7117=AXIS2_PLACEMENT_3D('',#10234,#8103,#8104);
#7118=AXIS2_PLACEMENT_3D('',#10235,#8105,#8106);
#7119=AXIS2_PLACEMENT_3D('',#10237,#8107,#8108);
#7120=AXIS2_PLACEMENT_3D('',#10240,#8110,#8111);
#7121=AXIS2_PLACEMENT_3D('',#10241,#8112,#8113);
#7122=AXIS2_PLACEMENT_3D('',#10243,#8114,#8115);
#7123=AXIS2_PLACEMENT_3D('',#10246,#8117,#8118);
#7124=AXIS2_PLACEMENT_3D('',#10247,#8119,#8120);
#7125=AXIS2_PLACEMENT_3D('',#10249,#8121,#8122);
#7126=AXIS2_PLACEMENT_3D('',#10252,#8124,#8125);
#7127=AXIS2_PLACEMENT_3D('',#10253,#8126,#8127);
#7128=AXIS2_PLACEMENT_3D('',#10255,#8128,#8129);
#7129=AXIS2_PLACEMENT_3D('',#10258,#8131,#8132);
#7130=AXIS2_PLACEMENT_3D('',#10259,#8133,#8134);
#7131=AXIS2_PLACEMENT_3D('',#10261,#8135,#8136);
#7132=AXIS2_PLACEMENT_3D('',#10264,#8138,#8139);
#7133=AXIS2_PLACEMENT_3D('',#10265,#8140,#8141);
#7134=AXIS2_PLACEMENT_3D('',#10267,#8142,#8143);
#7135=AXIS2_PLACEMENT_3D('',#10268,#8144,#8145);
#7136=AXIS2_PLACEMENT_3D('',#10270,#8146,#8147);
#7137=AXIS2_PLACEMENT_3D('',#10272,#8149,#8150);
#7138=AXIS2_PLACEMENT_3D('',#10274,#8151,#8152);
#7139=AXIS2_PLACEMENT_3D('',#10277,#8154,#8155);
#7140=AXIS2_PLACEMENT_3D('',#10278,#8156,#8157);
#7141=AXIS2_PLACEMENT_3D('',#10283,#8159,#8160);
#7142=AXIS2_PLACEMENT_3D('',#10286,#8162,#8163);
#7143=AXIS2_PLACEMENT_3D('',#10287,#8164,#8165);
#7144=AXIS2_PLACEMENT_3D('',#10303,#8173,#8174);
#7145=AXIS2_PLACEMENT_3D('',#10305,#8176,#8177);
#7146=AXIS2_PLACEMENT_3D('',#10309,#8180,#8181);
#7147=AXIS2_PLACEMENT_3D('',#10323,#8189,#8190);
#7148=AXIS2_PLACEMENT_3D('',#10329,#8194,#8195);
#7149=AXIS2_PLACEMENT_3D('',#10333,#8198,#8199);
#7150=AXIS2_PLACEMENT_3D('',#10337,#8202,#8203);
#7151=AXIS2_PLACEMENT_3D('',#10339,#8205,#8206);
#7152=AXIS2_PLACEMENT_3D('',#10343,#8209,#8210);
#7153=AXIS2_PLACEMENT_3D('',#10348,#8213,#8214);
#7154=AXIS2_PLACEMENT_3D('',#10349,#8215,#8216);
#7155=AXIS2_PLACEMENT_3D('',#10357,#8222,#8223);
#7156=AXIS2_PLACEMENT_3D('',#10358,#8224,#8225);
#7157=AXIS2_PLACEMENT_3D('',#10359,#8226,#8227);
#7158=AXIS2_PLACEMENT_3D('',#10361,#8229,#8230);
#7159=AXIS2_PLACEMENT_3D('',#10363,#8232,#8233);
#7160=AXIS2_PLACEMENT_3D('',#10364,#8234,#8235);
#8032=DIRECTION('axis',(0.,0.,1.));
#8033=DIRECTION('refdir',(1.,0.,0.));
#8034=DIRECTION('center_axis',(0.,1.,0.));
#8035=DIRECTION('ref_axis',(1.,0.,0.));
#8036=DIRECTION('center_axis',(0.,1.,0.));
#8037=DIRECTION('ref_axis',(1.,0.,0.));
#8038=DIRECTION('',(0.,1.,0.));
#8039=DIRECTION('center_axis',(0.,-1.,0.));
#8040=DIRECTION('ref_axis',(1.,0.,0.));
#8041=DIRECTION('center_axis',(0.,0.,1.));
#8042=DIRECTION('ref_axis',(1.,0.,0.));
#8043=DIRECTION('center_axis',(0.,0.,1.));
#8044=DIRECTION('ref_axis',(1.,0.,0.));
#8045=DIRECTION('',(0.,0.,1.));
#8046=DIRECTION('center_axis',(0.,0.,-1.));
#8047=DIRECTION('ref_axis',(1.,0.,0.));
#8048=DIRECTION('center_axis',(0.,0.,1.));
#8049=DIRECTION('ref_axis',(1.,0.,0.));
#8050=DIRECTION('center_axis',(0.,0.,1.));
#8051=DIRECTION('ref_axis',(1.,0.,0.));
#8052=DIRECTION('center_axis',(0.,0.,1.));
#8053=DIRECTION('ref_axis',(1.,0.,0.));
#8054=DIRECTION('',(0.,0.,1.));
#8055=DIRECTION('center_axis',(0.,0.,-1.));
#8056=DIRECTION('ref_axis',(1.,0.,0.));
#8057=DIRECTION('center_axis',(0.,0.,1.));
#8058=DIRECTION('ref_axis',(1.,0.,0.));
#8059=DIRECTION('center_axis',(0.,0.,1.));
#8060=DIRECTION('ref_axis',(1.,0.,0.));
#8061=DIRECTION('center_axis',(0.,0.,1.));
#8062=DIRECTION('ref_axis',(1.,0.,0.));
#8063=DIRECTION('',(0.,0.,1.));
#8064=DIRECTION('center_axis',(0.,0.,-1.));
#8065=DIRECTION('ref_axis',(1.,0.,0.));
#8066=DIRECTION('center_axis',(0.,0.,1.));
#8067=DIRECTION('ref_axis',(1.,0.,0.));
#8068=DIRECTION('center_axis',(0.,0.,1.));
#8069=DIRECTION('ref_axis',(1.,0.,0.));
#8070=DIRECTION('center_axis',(0.,0.,1.));
#8071=DIRECTION('ref_axis',(1.,0.,0.));
#8072=DIRECTION('',(0.,0.,1.));
#8073=DIRECTION('center_axis',(0.,0.,-1.));
#8074=DIRECTION('ref_axis',(1.,0.,0.));
#8075=DIRECTION('center_axis',(0.,0.,1.));
#8076=DIRECTION('ref_axis',(1.,0.,0.));
#8077=DIRECTION('center_axis',(0.,1.,0.));
#8078=DIRECTION('ref_axis',(1.,0.,0.));
#8079=DIRECTION('center_axis',(0.,1.,0.));
#8080=DIRECTION('ref_axis',(1.,0.,0.));
#8081=DIRECTION('',(0.,1.,0.));
#8082=DIRECTION('center_axis',(0.,-1.,0.));
#8083=DIRECTION('ref_axis',(1.,0.,0.));
#8084=DIRECTION('center_axis',(0.,1.,0.));
#8085=DIRECTION('ref_axis',(1.,0.,0.));
#8086=DIRECTION('center_axis',(0.,1.,0.));
#8087=DIRECTION('ref_axis',(1.,0.,0.));
#8088=DIRECTION('',(0.,1.,0.));
#8089=DIRECTION('center_axis',(0.,-1.,0.));
#8090=DIRECTION('ref_axis',(1.,0.,0.));
#8091=DIRECTION('center_axis',(0.,1.,0.));
#8092=DIRECTION('ref_axis',(1.,0.,0.));
#8093=DIRECTION('center_axis',(0.,1.,0.));
#8094=DIRECTION('ref_axis',(1.,0.,0.));
#8095=DIRECTION('',(0.,1.,0.));
#8096=DIRECTION('center_axis',(0.,-1.,0.));
#8097=DIRECTION('ref_axis',(1.,0.,0.));
#8098=DIRECTION('center_axis',(0.,1.,0.));
#8099=DIRECTION('ref_axis',(1.,0.,0.));
#8100=DIRECTION('center_axis',(0.,1.,0.));
#8101=DIRECTION('ref_axis',(1.,0.,0.));
#8102=DIRECTION('',(0.,1.,0.));
#8103=DIRECTION('center_axis',(0.,-1.,0.));
#8104=DIRECTION('ref_axis',(1.,0.,0.));
#8105=DIRECTION('center_axis',(0.,0.,1.));
#8106=DIRECTION('ref_axis',(1.,0.,0.));
#8107=DIRECTION('center_axis',(0.,0.,1.));
#8108=DIRECTION('ref_axis',(1.,0.,0.));
#8109=DIRECTION('',(0.,0.,1.));
#8110=DIRECTION('center_axis',(0.,0.,-1.));
#8111=DIRECTION('ref_axis',(1.,0.,0.));
#8112=DIRECTION('center_axis',(0.,0.,1.));
#8113=DIRECTION('ref_axis',(1.,0.,0.));
#8114=DIRECTION('center_axis',(0.,0.,1.));
#8115=DIRECTION('ref_axis',(1.,0.,0.));
#8116=DIRECTION('',(0.,0.,1.));
#8117=DIRECTION('center_axis',(0.,0.,-1.));
#8118=DIRECTION('ref_axis',(1.,0.,0.));
#8119=DIRECTION('center_axis',(0.,0.,1.));
#8120=DIRECTION('ref_axis',(1.,0.,0.));
#8121=DIRECTION('center_axis',(0.,0.,1.));
#8122=DIRECTION('ref_axis',(1.,0.,0.));
#8123=DIRECTION('',(0.,0.,1.));
#8124=DIRECTION('center_axis',(0.,0.,-1.));
#8125=DIRECTION('ref_axis',(1.,0.,0.));
#8126=DIRECTION('center_axis',(0.,0.,1.));
#8127=DIRECTION('ref_axis',(1.,0.,0.));
#8128=DIRECTION('center_axis',(0.,0.,1.));
#8129=DIRECTION('ref_axis',(1.,0.,0.));
#8130=DIRECTION('',(0.,0.,1.));
#8131=DIRECTION('center_axis',(0.,0.,-1.));
#8132=DIRECTION('ref_axis',(1.,0.,0.));
#8133=DIRECTION('center_axis',(0.,0.,1.));
#8134=DIRECTION('ref_axis',(1.,0.,0.));
#8135=DIRECTION('center_axis',(0.,0.,1.));
#8136=DIRECTION('ref_axis',(1.,0.,0.));
#8137=DIRECTION('',(0.,0.,1.));
#8138=DIRECTION('center_axis',(0.,0.,-1.));
#8139=DIRECTION('ref_axis',(1.,0.,0.));
#8140=DIRECTION('center_axis',(0.,0.,1.));
#8141=DIRECTION('ref_axis',(1.,0.,0.));
#8142=DIRECTION('center_axis',(0.,0.,1.));
#8143=DIRECTION('ref_axis',(1.,0.,0.));
#8144=DIRECTION('center_axis',(0.,0.,1.));
#8145=DIRECTION('ref_axis',(1.,0.,0.));
#8146=DIRECTION('center_axis',(0.,0.,1.));
#8147=DIRECTION('ref_axis',(1.,0.,0.));
#8148=DIRECTION('',(0.,0.,1.));
#8149=DIRECTION('center_axis',(0.,1.,0.));
#8150=DIRECTION('ref_axis',(1.,0.,0.));
#8151=DIRECTION('center_axis',(0.,1.,0.));
#8152=DIRECTION('ref_axis',(1.,0.,0.));
#8153=DIRECTION('',(0.,1.,0.));
#8154=DIRECTION('center_axis',(0.,-1.,0.));
#8155=DIRECTION('ref_axis',(1.,0.,0.));
#8156=DIRECTION('center_axis',(0.,0.,1.));
#8157=DIRECTION('ref_axis',(1.,0.,0.));
#8158=DIRECTION('',(0.,0.,1.));
#8159=DIRECTION('center_axis',(0.,0.,1.));
#8160=DIRECTION('ref_axis',(1.,0.,0.));
#8161=DIRECTION('',(0.,0.,-1.));
#8162=DIRECTION('center_axis',(0.,0.,1.));
#8163=DIRECTION('ref_axis',(1.,0.,0.));
#8164=DIRECTION('center_axis',(0.,-1.,0.));
#8165=DIRECTION('ref_axis',(1.,0.,0.));
#8166=DIRECTION('',(-1.,0.,0.));
#8167=DIRECTION('',(0.,0.,1.));
#8168=DIRECTION('',(1.,0.,0.));
#8169=DIRECTION('',(0.,0.,1.));
#8170=DIRECTION('',(1.,0.,0.));
#8171=DIRECTION('',(0.,0.,1.));
#8172=DIRECTION('',(1.,0.,0.));
#8173=DIRECTION('center_axis',(0.,1.,0.));
#8174=DIRECTION('ref_axis',(1.,0.,0.));
#8175=DIRECTION('',(1.,0.,0.));
#8176=DIRECTION('center_axis',(0.,0.,1.));
#8177=DIRECTION('ref_axis',(1.,0.,0.));
#8178=DIRECTION('',(1.,0.,0.));
#8179=DIRECTION('',(0.,1.,0.));
#8180=DIRECTION('center_axis',(0.,0.,1.));
#8181=DIRECTION('ref_axis',(1.,0.,0.));
#8182=DIRECTION('',(0.,-1.,0.));
#8183=DIRECTION('',(1.,0.,0.));
#8184=DIRECTION('',(0.,1.,0.));
#8185=DIRECTION('',(-1.,0.,0.));
#8186=DIRECTION('',(-1.,0.,0.));
#8187=DIRECTION('',(0.,1.,0.));
#8188=DIRECTION('',(0.,-1.,0.));
#8189=DIRECTION('center_axis',(0.,1.,0.));
#8190=DIRECTION('ref_axis',(-1.,0.,0.));
#8191=DIRECTION('',(-1.,0.,0.));
#8192=DIRECTION('',(0.,0.,1.));
#8193=DIRECTION('',(0.,0.,1.));
#8194=DIRECTION('center_axis',(1.,0.,0.));
#8195=DIRECTION('ref_axis',(0.,1.,0.));
#8196=DIRECTION('',(0.,1.,0.));
#8197=DIRECTION('',(0.,0.,1.));
#8198=DIRECTION('center_axis',(0.,-1.,0.));
#8199=DIRECTION('ref_axis',(1.,0.,0.));
#8200=DIRECTION('',(1.,0.,0.));
#8201=DIRECTION('',(0.,0.,1.));
#8202=DIRECTION('center_axis',(-1.,0.,0.));
#8203=DIRECTION('ref_axis',(0.,-1.,0.));
#8204=DIRECTION('',(0.,-1.,0.));
#8205=DIRECTION('center_axis',(1.,0.,0.));
#8206=DIRECTION('ref_axis',(0.,1.,0.));
#8207=DIRECTION('',(0.,0.,1.));
#8208=DIRECTION('',(0.,-1.,0.));
#8209=DIRECTION('center_axis',(0.,1.,0.));
#8210=DIRECTION('ref_axis',(6.12323399573677E-17,0.,-1.));
#8211=DIRECTION('',(0.,1.,0.));
#8212=DIRECTION('',(0.,-1.,0.));
#8213=DIRECTION('center_axis',(0.,1.,0.));
#8214=DIRECTION('ref_axis',(1.,0.,0.));
#8215=DIRECTION('center_axis',(0.,1.,0.));
#8216=DIRECTION('ref_axis',(-1.,0.,0.));
#8217=DIRECTION('',(-1.,0.,0.));
#8218=DIRECTION('',(-1.,0.,0.));
#8219=DIRECTION('',(0.,0.,1.));
#8220=DIRECTION('',(-1.,0.,0.));
#8221=DIRECTION('',(0.,0.,1.));
#8222=DIRECTION('center_axis',(0.,0.,-1.));
#8223=DIRECTION('ref_axis',(-1.,0.,0.));
#8224=DIRECTION('center_axis',(0.,0.,-1.));
#8225=DIRECTION('ref_axis',(-1.,0.,0.));
#8226=DIRECTION('center_axis',(1.,0.,0.));
#8227=DIRECTION('ref_axis',(0.,1.,0.));
#8228=DIRECTION('',(0.,1.,0.));
#8229=DIRECTION('center_axis',(-1.,0.,0.));
#8230=DIRECTION('ref_axis',(0.,-1.,0.));
#8231=DIRECTION('',(0.,-1.,0.));
#8232=DIRECTION('center_axis',(0.,0.,1.));
#8233=DIRECTION('ref_axis',(1.,0.,0.));
#8234=DIRECTION('center_axis',(0.,0.,1.));
#8235=DIRECTION('ref_axis',(1.,0.,0.));
#10176=CARTESIAN_POINT('',(0.,0.,0.));
#10177=CARTESIAN_POINT('Origin',(-5.25982293614231,-0.9,14.8604204653858));
#10178=CARTESIAN_POINT('',(-5.48482293614231,-0.8,14.8604204653858));
#10179=CARTESIAN_POINT('Origin',(-5.25982293614231,-0.8,14.8604204653858));
#10180=CARTESIAN_POINT('',(-5.48482293614231,0.8,14.8604204653858));
#10181=CARTESIAN_POINT('',(-5.48482293614231,-0.9,14.8604204653858));
#10182=CARTESIAN_POINT('Origin',(-5.25982293614231,0.8,14.8604204653858));
#10183=CARTESIAN_POINT('Origin',(-1.13137084989848,-1.13137084989848,15.8));
#10184=CARTESIAN_POINT('',(-1.29637084989848,-1.13137084989848,15.8));
#10185=CARTESIAN_POINT('Origin',(-1.13137084989848,-1.13137084989848,15.8));
#10186=CARTESIAN_POINT('',(-1.29637084989848,-1.13137084989848,16.5));
#10187=CARTESIAN_POINT('',(-1.29637084989848,-1.13137084989848,15.8));
#10188=CARTESIAN_POINT('Origin',(-1.13137084989848,-1.13137084989848,16.5));
#10189=CARTESIAN_POINT('Origin',(-1.13137084989848,-1.13137084989848,15.8));
#10190=CARTESIAN_POINT('Origin',(-1.13137084989848,1.13137084989848,15.8));
#10191=CARTESIAN_POINT('',(-1.29637084989848,1.13137084989848,15.8));
#10192=CARTESIAN_POINT('Origin',(-1.13137084989848,1.13137084989848,15.8));
#10193=CARTESIAN_POINT('',(-1.29637084989848,1.13137084989848,16.5));
#10194=CARTESIAN_POINT('',(-1.29637084989848,1.13137084989848,15.8));
#10195=CARTESIAN_POINT('Origin',(-1.13137084989848,1.13137084989848,16.5));
#10196=CARTESIAN_POINT('Origin',(-1.13137084989848,1.13137084989848,15.8));
#10197=CARTESIAN_POINT('Origin',(1.13137084989848,1.13137084989848,15.8));
#10198=CARTESIAN_POINT('',(0.966370849898476,1.13137084989848,15.8));
#10199=CARTESIAN_POINT('Origin',(1.13137084989848,1.13137084989848,15.8));
#10200=CARTESIAN_POINT('',(0.966370849898476,1.13137084989848,16.5));
#10201=CARTESIAN_POINT('',(0.966370849898476,1.13137084989848,15.8));
#10202=CARTESIAN_POINT('Origin',(1.13137084989848,1.13137084989848,16.5));
#10203=CARTESIAN_POINT('Origin',(1.13137084989848,1.13137084989848,15.8));
#10204=CARTESIAN_POINT('Origin',(1.13137084989848,-1.13137084989848,15.8));
#10205=CARTESIAN_POINT('',(0.966370849898476,-1.13137084989848,15.8));
#10206=CARTESIAN_POINT('Origin',(1.13137084989848,-1.13137084989848,15.8));
#10207=CARTESIAN_POINT('',(0.966370849898476,-1.13137084989848,16.5));
#10208=CARTESIAN_POINT('',(0.966370849898476,-1.13137084989848,15.8));
#10209=CARTESIAN_POINT('Origin',(1.13137084989848,-1.13137084989848,16.5));
#10210=CARTESIAN_POINT('Origin',(1.13137084989848,-1.13137084989848,15.8));
#10211=CARTESIAN_POINT('Origin',(-5.23743686707646,-0.9,9.76256313292354));
#10212=CARTESIAN_POINT('',(-5.40243686707646,-0.8,9.76256313292354));
#10213=CARTESIAN_POINT('Origin',(-5.23743686707646,-0.8,9.76256313292354));
#10214=CARTESIAN_POINT('',(-5.40243686707646,0.8,9.76256313292354));
#10215=CARTESIAN_POINT('',(-5.40243686707646,-0.9,9.76256313292354));
#10216=CARTESIAN_POINT('Origin',(-5.23743686707646,0.8,9.76256313292354));
#10217=CARTESIAN_POINT('Origin',(-5.23743686707646,-0.9,12.2374368670765));
#10218=CARTESIAN_POINT('',(-5.40243686707646,-0.8,12.2374368670765));
#10219=CARTESIAN_POINT('Origin',(-5.23743686707646,-0.8,12.2374368670765));
#10220=CARTESIAN_POINT('',(-5.40243686707646,0.8,12.2374368670765));
#10221=CARTESIAN_POINT('',(-5.40243686707646,-0.9,12.2374368670765));
#10222=CARTESIAN_POINT('Origin',(-5.23743686707646,0.8,12.2374368670765));
#10223=CARTESIAN_POINT('Origin',(-2.76256313292354,-0.9,12.2374368670765));
#10224=CARTESIAN_POINT('',(-2.92756313292354,-0.8,12.2374368670765));
#10225=CARTESIAN_POINT('Origin',(-2.76256313292354,-0.8,12.2374368670765));
#10226=CARTESIAN_POINT('',(-2.92756313292354,0.8,12.2374368670765));
#10227=CARTESIAN_POINT('',(-2.92756313292354,-0.9,12.2374368670765));
#10228=CARTESIAN_POINT('Origin',(-2.76256313292354,0.8,12.2374368670765));
#10229=CARTESIAN_POINT('Origin',(-2.76256313292354,-0.9,9.76256313292354));
#10230=CARTESIAN_POINT('',(-2.92756313292354,-0.8,9.76256313292354));
#10231=CARTESIAN_POINT('Origin',(-2.76256313292354,-0.8,9.76256313292354));
#10232=CARTESIAN_POINT('',(-2.92756313292354,0.8,9.76256313292354));
#10233=CARTESIAN_POINT('',(-2.92756313292354,-0.9,9.76256313292354));
#10234=CARTESIAN_POINT('Origin',(-2.76256313292354,0.8,9.76256313292354));
#10235=CARTESIAN_POINT('Origin',(-6.,-1.4,0.9));
#10236=CARTESIAN_POINT('',(-6.275,-1.4,1.));
#10237=CARTESIAN_POINT('Origin',(-6.,-1.4,1.));
#10238=CARTESIAN_POINT('',(-6.275,-1.4,1.8));
#10239=CARTESIAN_POINT('',(-6.275,-1.4,0.9));
#10240=CARTESIAN_POINT('Origin',(-6.,-1.4,1.8));
#10241=CARTESIAN_POINT('Origin',(-8.5,1.4,0.9));
#10242=CARTESIAN_POINT('',(-8.775,1.4,1.));
#10243=CARTESIAN_POINT('Origin',(-8.5,1.4,1.));
#10244=CARTESIAN_POINT('',(-8.775,1.4,1.8));
#10245=CARTESIAN_POINT('',(-8.775,1.4,0.9));
#10246=CARTESIAN_POINT('Origin',(-8.5,1.4,1.8));
#10247=CARTESIAN_POINT('Origin',(-8.5,-1.4,0.9));
#10248=CARTESIAN_POINT('',(-8.775,-1.4,1.));
#10249=CARTESIAN_POINT('Origin',(-8.5,-1.4,1.));
#10250=CARTESIAN_POINT('',(-8.775,-1.4,1.8));
#10251=CARTESIAN_POINT('',(-8.775,-1.4,0.9));
#10252=CARTESIAN_POINT('Origin',(-8.5,-1.4,1.8));
#10253=CARTESIAN_POINT('Origin',(-6.,1.4,0.9));
#10254=CARTESIAN_POINT('',(-6.275,1.4,1.));
#10255=CARTESIAN_POINT('Origin',(-6.,1.4,1.));
#10256=CARTESIAN_POINT('',(-6.275,1.4,1.8));
#10257=CARTESIAN_POINT('',(-6.275,1.4,0.9));
#10258=CARTESIAN_POINT('Origin',(-6.,1.4,1.8));
#10259=CARTESIAN_POINT('Origin',(0.,0.,12.5));
#10260=CARTESIAN_POINT('',(-1.05,-1.28587913910472E-16,12.5));
#10261=CARTESIAN_POINT('Origin',(0.,0.,12.5));
#10262=CARTESIAN_POINT('',(-1.05,1.28587913910472E-16,16.5));
#10263=CARTESIAN_POINT('',(-1.05,-1.28587913910472E-16,12.5));
#10264=CARTESIAN_POINT('Origin',(0.,0.,16.5));
#10265=CARTESIAN_POINT('Origin',(0.,0.,12.5));
#10266=CARTESIAN_POINT('',(-0.625,-7.65404249467096E-17,12.5));
#10267=CARTESIAN_POINT('Origin',(0.,0.,12.5));
#10268=CARTESIAN_POINT('Origin',(0.,0.,11.9));
#10269=CARTESIAN_POINT('',(-0.625,-7.65404249467096E-17,12.));
#10270=CARTESIAN_POINT('Origin',(0.,0.,12.));
#10271=CARTESIAN_POINT('',(-0.625,-7.65404249467096E-17,11.9));
#10272=CARTESIAN_POINT('Origin',(-4.,-0.9,11.));
#10273=CARTESIAN_POINT('',(-5.5,-0.8,11.));
#10274=CARTESIAN_POINT('Origin',(-4.,-0.8,11.));
#10275=CARTESIAN_POINT('',(-5.5,0.8,11.));
#10276=CARTESIAN_POINT('',(-5.5,-0.9,11.));
#10277=CARTESIAN_POINT('Origin',(-4.,0.8,11.));
#10278=CARTESIAN_POINT('Origin',(0.,0.,12.));
#10279=CARTESIAN_POINT('',(-1.83303027798234,-0.8,12.));
#10280=CARTESIAN_POINT('',(-1.83303027798234,-0.8,16.5));
#10281=CARTESIAN_POINT('',(-1.83303027798234,-0.8,12.));
#10282=CARTESIAN_POINT('',(-1.83303027798234,0.8,12.));
#10283=CARTESIAN_POINT('Origin',(0.,0.,12.));
#10284=CARTESIAN_POINT('',(-1.83303027798234,0.8,16.5));
#10285=CARTESIAN_POINT('',(-1.83303027798234,0.8,12.));
#10286=CARTESIAN_POINT('Origin',(0.,0.,16.5));
#10287=CARTESIAN_POINT('Origin',(-8.,-0.8,1.));
#10288=CARTESIAN_POINT('',(-6.5,-0.8,16.5));
#10289=CARTESIAN_POINT('',(1.5,-0.8,16.5));
#10290=CARTESIAN_POINT('',(-6.5,-0.8,17.5));
#10291=CARTESIAN_POINT('',(-6.5,-0.8,1.));
#10292=CARTESIAN_POINT('',(-8.,-0.8,17.5));
#10293=CARTESIAN_POINT('',(-8.,-0.8,17.5));
#10294=CARTESIAN_POINT('',(-8.,-0.8,1.8));
#10295=CARTESIAN_POINT('',(-8.,-0.8,1.));
#10296=CARTESIAN_POINT('',(-6.5,-0.8,1.8));
#10297=CARTESIAN_POINT('',(-7.625,-0.8,1.8));
#10298=CARTESIAN_POINT('',(-6.5,-0.8,12.));
#10299=CARTESIAN_POINT('',(-6.5,-0.8,1.));
#10300=CARTESIAN_POINT('',(-5.95959179422654,-0.8,12.));
#10301=CARTESIAN_POINT('',(-8.,-0.8,12.));
#10302=CARTESIAN_POINT('',(-2.04040820577346,-0.8,12.));
#10303=CARTESIAN_POINT('Origin',(-4.,-0.8,11.));
#10304=CARTESIAN_POINT('',(-8.,-0.8,12.));
#10305=CARTESIAN_POINT('Origin',(-8.,-0.8,16.5));
#10306=CARTESIAN_POINT('',(-6.5,0.8,16.5));
#10307=CARTESIAN_POINT('',(1.5,0.8,16.5));
#10308=CARTESIAN_POINT('',(-6.5,-0.8,16.5));
#10309=CARTESIAN_POINT('Origin',(-7.25,0.,1.8));
#10310=CARTESIAN_POINT('',(-9.,2.,1.8));
#10311=CARTESIAN_POINT('',(-9.,-2.,1.8));
#10312=CARTESIAN_POINT('',(-9.,2.,1.8));
#10313=CARTESIAN_POINT('',(-5.5,-2.,1.8));
#10314=CARTESIAN_POINT('',(-9.,-2.,1.8));
#10315=CARTESIAN_POINT('',(-5.5,2.,1.8));
#10316=CARTESIAN_POINT('',(-5.5,-2.,1.8));
#10317=CARTESIAN_POINT('',(-5.5,2.,1.8));
#10318=CARTESIAN_POINT('',(-6.5,0.8,1.8));
#10319=CARTESIAN_POINT('',(-8.,0.8,1.8));
#10320=CARTESIAN_POINT('',(-6.875,0.8,1.8));
#10321=CARTESIAN_POINT('',(-6.5,-0.4,1.8));
#10322=CARTESIAN_POINT('',(-8.,0.4,1.8));
#10323=CARTESIAN_POINT('Origin',(-5.5,2.,1.));
#10324=CARTESIAN_POINT('',(-5.5,2.,1.));
#10325=CARTESIAN_POINT('',(-9.,2.,1.));
#10326=CARTESIAN_POINT('',(-5.5,2.,1.));
#10327=CARTESIAN_POINT('',(-9.,2.,1.));
#10328=CARTESIAN_POINT('',(-5.5,2.,1.));
#10329=CARTESIAN_POINT('Origin',(-5.5,-2.,1.));
#10330=CARTESIAN_POINT('',(-5.5,-2.,1.));
#10331=CARTESIAN_POINT('',(-5.5,-2.,1.));
#10332=CARTESIAN_POINT('',(-5.5,-2.,1.));
#10333=CARTESIAN_POINT('Origin',(-9.,-2.,1.));
#10334=CARTESIAN_POINT('',(-9.,-2.,1.));
#10335=CARTESIAN_POINT('',(-9.,-2.,1.));
#10336=CARTESIAN_POINT('',(-9.,-2.,1.));
#10337=CARTESIAN_POINT('Origin',(-9.,2.,1.));
#10338=CARTESIAN_POINT('',(-9.,2.,1.));
#10339=CARTESIAN_POINT('Origin',(-6.5,-0.8,1.));
#10340=CARTESIAN_POINT('',(-6.5,0.8,12.));
#10341=CARTESIAN_POINT('',(-6.5,0.8,1.));
#10342=CARTESIAN_POINT('',(-6.5,-0.8,12.));
#10343=CARTESIAN_POINT('Origin',(-4.,-0.8,11.));
#10344=CARTESIAN_POINT('',(-2.04040820577346,0.8,12.));
#10345=CARTESIAN_POINT('',(-2.04040820577346,-0.8,12.));
#10346=CARTESIAN_POINT('',(-5.95959179422654,0.8,12.));
#10347=CARTESIAN_POINT('',(-5.95959179422654,-0.8,12.));
#10348=CARTESIAN_POINT('Origin',(-4.,0.8,11.));
#10349=CARTESIAN_POINT('Origin',(-6.5,0.8,1.));
#10350=CARTESIAN_POINT('',(-8.,0.8,12.));
#10351=CARTESIAN_POINT('',(-8.,0.8,12.));
#10352=CARTESIAN_POINT('',(-8.,0.8,17.5));
#10353=CARTESIAN_POINT('',(-8.,0.8,1.));
#10354=CARTESIAN_POINT('',(-6.5,0.8,17.5));
#10355=CARTESIAN_POINT('',(-6.5,0.8,17.5));
#10356=CARTESIAN_POINT('',(-6.5,0.8,1.));
#10357=CARTESIAN_POINT('Origin',(1.5,-0.8,12.));
#10358=CARTESIAN_POINT('Origin',(1.5,-0.8,12.));
#10359=CARTESIAN_POINT('Origin',(-6.5,-0.8,1.));
#10360=CARTESIAN_POINT('',(-6.5,-0.8,17.5));
#10361=CARTESIAN_POINT('Origin',(-8.,0.8,1.));
#10362=CARTESIAN_POINT('',(-8.,0.8,17.5));
#10363=CARTESIAN_POINT('Origin',(-7.25,0.,17.5));
#10364=CARTESIAN_POINT('Origin',(-7.25,0.,1.));
#12327=UNCERTAINTY_MEASURE_WITH_UNIT(LENGTH_MEASURE(0.001),#12414,
'DISTANCE_ACCURACY_VALUE',
'Maximum model space distance between geometric entities at asserted c
onnectivities');
#12367=UNCERTAINTY_MEASURE_WITH_UNIT(LENGTH_MEASURE(0.001),#12414,
'DISTANCE_ACCURACY_VALUE',
'Maximum model space distance between geometric entities at asserted c
onnectivities');
#12373=(
GEOMETRIC_REPRESENTATION_CONTEXT(3)
GLOBAL_UNCERTAINTY_ASSIGNED_CONTEXT((#12327))
GLOBAL_UNIT_ASSIGNED_CONTEXT((#12414,#12416,#12417))
REPRESENTATION_CONTEXT('','3D')
);
#12413=(
GEOMETRIC_REPRESENTATION_CONTEXT(3)
GLOBAL_UNCERTAINTY_ASSIGNED_CONTEXT((#12367))
GLOBAL_UNIT_ASSIGNED_CONTEXT((#12414,#12416,#12417))
REPRESENTATION_CONTEXT('','3D')
);
#12414=(
LENGTH_UNIT()
NAMED_UNIT(*)
SI_UNIT(.CENTI.,.METRE.)
);
#12416=(
NAMED_UNIT(*)
PLANE_ANGLE_UNIT()
SI_UNIT($,.RADIAN.)
);
#12417=(
NAMED_UNIT(*)
SI_UNIT($,.STERADIAN.)
SOLID_ANGLE_UNIT()
);
#12423=SHAPE_DEFINITION_REPRESENTATION(#12468,#12576);
#12468=PRODUCT_DEFINITION_SHAPE('',$,#12622);
#12576=SHAPE_REPRESENTATION('',(#7086),#12373);
#12616=PRODUCT_DEFINITION_CONTEXT('part definition',#12753,'design');
#12622=PRODUCT_DEFINITION('Bearing frame','Bearing frame',#12667,#12616);
#12667=PRODUCT_DEFINITION_FORMATION('',$,#12760);
#12753=APPLICATION_CONTEXT(
'Core Data for Automotive Mechanical Design Process');
#12754=PRODUCT_CONTEXT('part definition',#12753,'mechanical');
#12760=PRODUCT('Bearing frame','Bearing frame','Bearing frame',(#12754));
#12863=COLOUR_RGB('Grey',0.48,0.52,0.57);
#12864=FILL_AREA_STYLE_COLOUR('',#12863);
#12865=FILL_AREA_STYLE('',(#12864));
#12866=SURFACE_STYLE_FILL_AREA(#12865);
#12867=SURFACE_SIDE_STYLE('',(#12866));
#12868=SURFACE_STYLE_USAGE(.BOTH.,#12867);
#12869=PRESENTATION_STYLE_ASSIGNMENT((#12868));
ENDSEC;
END-ISO-10303-21;
